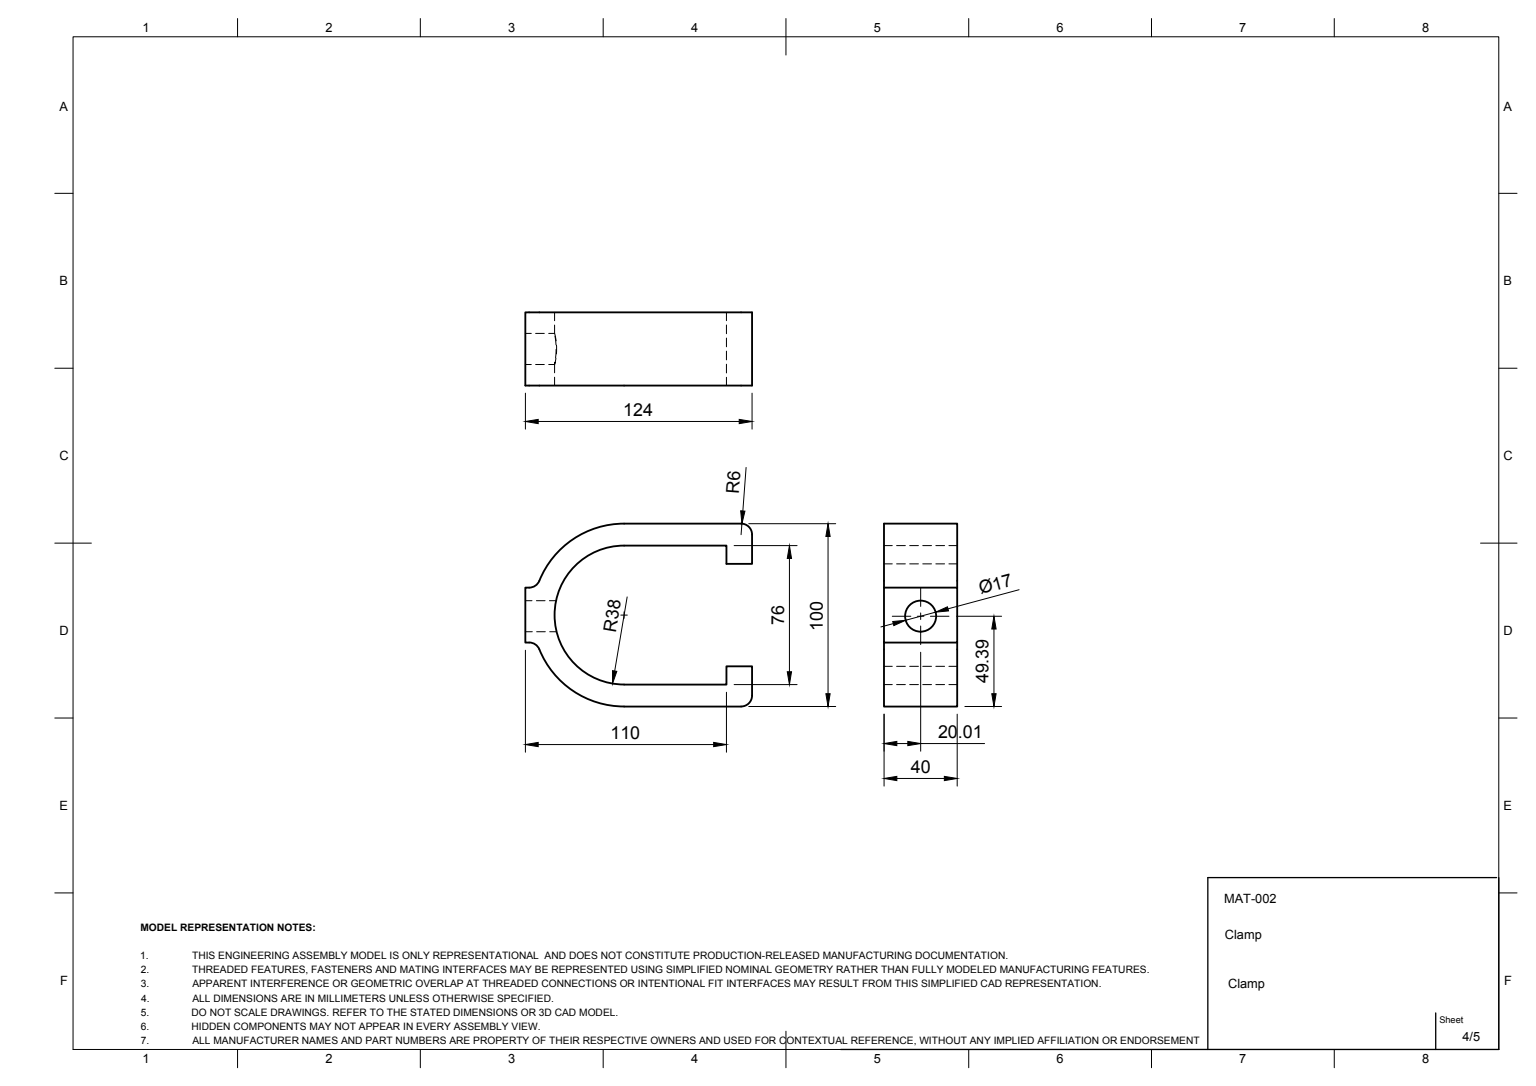
ISO-10303-21;
HEADER;
/* Generated by software containing ST-Developer
 * from STEP Tools, Inc. (www.steptools.com) 
 */

FILE_DESCRIPTION(
/* description */ ('STEP AP214'),
/* implementation_level */ '2;1');

FILE_NAME(
/* name */ 'Clamp.step',
/* time_stamp */ '2026-11-14T04:35:10-08:00',
/* author */ (''),
/* organization */ (''),
/* preprocessor_version */ 'ST-DEVELOPER v20.2',
/* originating_system */ 'Autodesk Translation Framework v15.17.0.0',
/* authorisation */ '');

FILE_SCHEMA (('AUTOMOTIVE_DESIGN { 1 0 10303 214 3 1 1 }'));
ENDSEC;

DATA;
#10=MECHANICAL_DESIGN_GEOMETRIC_PRESENTATION_REPRESENTATION('',(#108),#2477);
#47=FACE_BOUND('',#226,.T.);
#48=FACE_BOUND('',#235,.T.);
#50=CIRCLE('',#1508,8.49999999999998);
#51=CIRCLE('',#1512,38.);
#52=CIRCLE('',#1513,38.);
#53=CIRCLE('',#1520,50.);
#54=CIRCLE('',#1521,50.);
#55=CIRCLE('',#1526,50.);
#56=CIRCLE('',#1527,50.);
#57=CIRCLE('',#1532,6.);
#58=CIRCLE('',#1533,6.);
#59=CIRCLE('',#1534,6.);
#60=CIRCLE('',#1535,6.);
#61=CIRCLE('',#1537,6.);
#62=CIRCLE('',#1538,6.);
#63=CIRCLE('',#1539,6.);
#64=CIRCLE('',#1540,6.);
#86=B_SPLINE_CURVE_WITH_KNOTS('',3,(#2159,#2160,#2161,#2162,#2163,#2164,
#2165,#2166,#2167,#2168,#2169,#2170,#2171,#2172,#2173,#2174,#2175,#2176,
#2177),.UNSPECIFIED.,.F.,.F.,(4,2,2,2,3,2,2,2,4),(3.85552474626411,4.17737028900463,
4.49921583174514,4.82064221776852,5.14206860379189,5.46349498981527,5.78492137583865,
6.10676691857916,6.42861246131968),.UNSPECIFIED.);
#87=B_SPLINE_CURVE_WITH_KNOTS('',3,(#2181,#2182,#2183,#2184,#2185,#2186,
#2187,#2188,#2189,#2190,#2191,#2192,#2193,#2194,#2195,#2196,#2197,#2198),
 .UNSPECIFIED.,.F.,.F.,(4,2,2,2,2,2,2,2,4),(6.42861246131968,6.74954370836776,
7.07047495541584,7.39178893055184,7.71310290568784,8.03441688082384,8.35573085595985,
8.67666210300793,8.99759335005601),.UNSPECIFIED.);
#88=CYLINDRICAL_SURFACE('',#1507,8.49999999999998);
#89=CYLINDRICAL_SURFACE('',#1511,38.);
#90=CYLINDRICAL_SURFACE('',#1519,50.);
#91=CYLINDRICAL_SURFACE('',#1525,50.);
#92=CYLINDRICAL_SURFACE('',#1541,6.);
#93=CYLINDRICAL_SURFACE('',#1542,6.);
#94=CYLINDRICAL_SURFACE('',#1543,6.);
#95=CYLINDRICAL_SURFACE('',#1544,6.);
#100=SHAPE_REPRESENTATION_RELATIONSHIP('SRR','None',#2498,#104);
#104=ADVANCED_BREP_SHAPE_REPRESENTATION('',(#112),#2474);
#108=STYLED_ITEM('',(#2527),#112);
#112=MANIFOLD_SOLID_BREP('Body1',#1428);
#143=FACE_OUTER_BOUND('',#222,.T.);
#144=FACE_OUTER_BOUND('',#223,.T.);
#145=FACE_OUTER_BOUND('',#224,.T.);
#146=FACE_OUTER_BOUND('',#225,.T.);
#147=FACE_OUTER_BOUND('',#227,.T.);
#148=FACE_OUTER_BOUND('',#228,.T.);
#149=FACE_OUTER_BOUND('',#229,.T.);
#150=FACE_OUTER_BOUND('',#230,.T.);
#151=FACE_OUTER_BOUND('',#231,.T.);
#152=FACE_OUTER_BOUND('',#232,.T.);
#153=FACE_OUTER_BOUND('',#233,.T.);
#154=FACE_OUTER_BOUND('',#234,.T.);
#155=FACE_OUTER_BOUND('',#236,.T.);
#156=FACE_OUTER_BOUND('',#237,.T.);
#157=FACE_OUTER_BOUND('',#238,.T.);
#158=FACE_OUTER_BOUND('',#239,.T.);
#159=FACE_OUTER_BOUND('',#240,.T.);
#160=FACE_OUTER_BOUND('',#241,.T.);
#161=FACE_OUTER_BOUND('',#242,.T.);
#162=FACE_OUTER_BOUND('',#243,.T.);
#163=FACE_OUTER_BOUND('',#244,.T.);
#164=FACE_OUTER_BOUND('',#245,.T.);
#165=FACE_OUTER_BOUND('',#246,.T.);
#222=EDGE_LOOP('',(#1050,#1051,#1052,#1053,#1054));
#223=EDGE_LOOP('',(#1055,#1056,#1057,#1058));
#224=EDGE_LOOP('',(#1059,#1060,#1061,#1062));
#225=EDGE_LOOP('',(#1063,#1064,#1065,#1066));
#226=EDGE_LOOP('',(#1067,#1068));
#227=EDGE_LOOP('',(#1069,#1070,#1071,#1072));
#228=EDGE_LOOP('',(#1073,#1074,#1075,#1076));
#229=EDGE_LOOP('',(#1077,#1078,#1079,#1080));
#230=EDGE_LOOP('',(#1081,#1082,#1083,#1084));
#231=EDGE_LOOP('',(#1085,#1086,#1087,#1088));
#232=EDGE_LOOP('',(#1089,#1090,#1091,#1092));
#233=EDGE_LOOP('',(#1093,#1094,#1095,#1096));
#234=EDGE_LOOP('',(#1097,#1098,#1099,#1100));
#235=EDGE_LOOP('',(#1101));
#236=EDGE_LOOP('',(#1102,#1103,#1104,#1105));
#237=EDGE_LOOP('',(#1106,#1107,#1108,#1109));
#238=EDGE_LOOP('',(#1110,#1111,#1112,#1113));
#239=EDGE_LOOP('',(#1114,#1115,#1116,#1117));
#240=EDGE_LOOP('',(#1118,#1119,#1120,#1121));
#241=EDGE_LOOP('',(#1122,#1123,#1124,#1125,#1126,#1127,#1128,#1129,#1130,
#1131,#1132,#1133,#1134,#1135,#1136,#1137,#1138,#1139,#1140,#1141));
#242=EDGE_LOOP('',(#1142,#1143,#1144,#1145,#1146,#1147,#1148,#1149,#1150,
#1151,#1152,#1153,#1154,#1155,#1156,#1157,#1158,#1159,#1160,#1161));
#243=EDGE_LOOP('',(#1162,#1163,#1164,#1165));
#244=EDGE_LOOP('',(#1166,#1167,#1168,#1169));
#245=EDGE_LOOP('',(#1170,#1171,#1172,#1173));
#246=EDGE_LOOP('',(#1174,#1175,#1176,#1177));
#354=LINE('',#2179,#501);
#355=LINE('',#2202,#502);
#356=LINE('',#2204,#503);
#357=LINE('',#2206,#504);
#358=LINE('',#2207,#505);
#359=LINE('',#2210,#506);
#360=LINE('',#2212,#507);
#361=LINE('',#2213,#508);
#362=LINE('',#2218,#509);
#363=LINE('',#2222,#510);
#364=LINE('',#2224,#511);
#365=LINE('',#2225,#512);
#366=LINE('',#2228,#513);
#367=LINE('',#2230,#514);
#368=LINE('',#2231,#515);
#369=LINE('',#2234,#516);
#370=LINE('',#2236,#517);
#371=LINE('',#2237,#518);
#372=LINE('',#2240,#519);
#373=LINE('',#2242,#520);
#374=LINE('',#2243,#521);
#375=LINE('',#2247,#522);
#376=LINE('',#2249,#523);
#377=LINE('',#2251,#524);
#378=LINE('',#2252,#525);
#379=LINE('',#2257,#526);
#380=LINE('',#2262,#527);
#381=LINE('',#2264,#528);
#382=LINE('',#2266,#529);
#383=LINE('',#2267,#530);
#384=LINE('',#2270,#531);
#385=LINE('',#2272,#532);
#386=LINE('',#2273,#533);
#387=LINE('',#2276,#534);
#388=LINE('',#2278,#535);
#389=LINE('',#2279,#536);
#390=LINE('',#2285,#537);
#391=LINE('',#2288,#538);
#392=LINE('',#2291,#539);
#393=LINE('',#2293,#540);
#394=LINE('',#2294,#541);
#395=LINE('',#2298,#542);
#396=LINE('',#2300,#543);
#397=LINE('',#2302,#544);
#398=LINE('',#2303,#545);
#399=LINE('',#2305,#546);
#400=LINE('',#2306,#547);
#501=VECTOR('',#1742,8.49999999999998);
#502=VECTOR('',#1747,1000.);
#503=VECTOR('',#1748,1000.);
#504=VECTOR('',#1749,1000.);
#505=VECTOR('',#1750,1000.);
#506=VECTOR('',#1753,1000.);
#507=VECTOR('',#1754,1000.);
#508=VECTOR('',#1755,1000.);
#509=VECTOR('',#1760,1000.);
#510=VECTOR('',#1765,1000.);
#511=VECTOR('',#1766,1000.);
#512=VECTOR('',#1767,1000.);
#513=VECTOR('',#1770,1000.);
#514=VECTOR('',#1771,1000.);
#515=VECTOR('',#1772,1000.);
#516=VECTOR('',#1775,1000.);
#517=VECTOR('',#1776,1000.);
#518=VECTOR('',#1777,1000.);
#519=VECTOR('',#1780,1000.);
#520=VECTOR('',#1781,1000.);
#521=VECTOR('',#1782,1000.);
#522=VECTOR('',#1785,1000.);
#523=VECTOR('',#1786,1000.);
#524=VECTOR('',#1787,1000.);
#525=VECTOR('',#1788,1000.);
#526=VECTOR('',#1793,1000.);
#527=VECTOR('',#1798,1000.);
#528=VECTOR('',#1799,1000.);
#529=VECTOR('',#1800,1000.);
#530=VECTOR('',#1801,1000.);
#531=VECTOR('',#1804,1000.);
#532=VECTOR('',#1805,1000.);
#533=VECTOR('',#1806,1000.);
#534=VECTOR('',#1809,1000.);
#535=VECTOR('',#1810,1000.);
#536=VECTOR('',#1811,1000.);
#537=VECTOR('',#1816,1000.);
#538=VECTOR('',#1819,1000.);
#539=VECTOR('',#1822,1000.);
#540=VECTOR('',#1823,1000.);
#541=VECTOR('',#1824,1000.);
#542=VECTOR('',#1827,1000.);
#543=VECTOR('',#1828,1000.);
#544=VECTOR('',#1829,1000.);
#545=VECTOR('',#1830,1000.);
#546=VECTOR('',#1833,1000.);
#547=VECTOR('',#1834,1000.);
#622=VERTEX_POINT('',#2157);
#623=VERTEX_POINT('',#2158);
#624=VERTEX_POINT('',#2178);
#625=VERTEX_POINT('',#2200);
#626=VERTEX_POINT('',#2201);
#627=VERTEX_POINT('',#2203);
#628=VERTEX_POINT('',#2205);
#629=VERTEX_POINT('',#2209);
#630=VERTEX_POINT('',#2211);
#631=VERTEX_POINT('',#2215);
#632=VERTEX_POINT('',#2217);
#633=VERTEX_POINT('',#2221);
#634=VERTEX_POINT('',#2223);
#635=VERTEX_POINT('',#2227);
#636=VERTEX_POINT('',#2229);
#637=VERTEX_POINT('',#2233);
#638=VERTEX_POINT('',#2235);
#639=VERTEX_POINT('',#2239);
#640=VERTEX_POINT('',#2241);
#641=VERTEX_POINT('',#2245);
#642=VERTEX_POINT('',#2246);
#643=VERTEX_POINT('',#2248);
#644=VERTEX_POINT('',#2250);
#645=VERTEX_POINT('',#2254);
#646=VERTEX_POINT('',#2256);
#647=VERTEX_POINT('',#2260);
#648=VERTEX_POINT('',#2261);
#649=VERTEX_POINT('',#2263);
#650=VERTEX_POINT('',#2265);
#651=VERTEX_POINT('',#2269);
#652=VERTEX_POINT('',#2271);
#653=VERTEX_POINT('',#2275);
#654=VERTEX_POINT('',#2277);
#655=VERTEX_POINT('',#2281);
#656=VERTEX_POINT('',#2282);
#657=VERTEX_POINT('',#2284);
#658=VERTEX_POINT('',#2286);
#659=VERTEX_POINT('',#2290);
#660=VERTEX_POINT('',#2292);
#661=VERTEX_POINT('',#2296);
#662=VERTEX_POINT('',#2297);
#663=VERTEX_POINT('',#2299);
#664=VERTEX_POINT('',#2301);
#775=EDGE_CURVE('',#622,#623,#86,.T.);
#776=EDGE_CURVE('',#623,#624,#354,.T.);
#777=EDGE_CURVE('',#624,#624,#50,.T.);
#778=EDGE_CURVE('',#623,#622,#87,.T.);
#779=EDGE_CURVE('',#625,#626,#355,.T.);
#780=EDGE_CURVE('',#627,#625,#356,.T.);
#781=EDGE_CURVE('',#627,#628,#357,.T.);
#782=EDGE_CURVE('',#628,#626,#358,.T.);
#783=EDGE_CURVE('',#629,#625,#359,.T.);
#784=EDGE_CURVE('',#630,#629,#360,.T.);
#785=EDGE_CURVE('',#630,#627,#361,.T.);
#786=EDGE_CURVE('',#631,#629,#51,.T.);
#787=EDGE_CURVE('',#632,#631,#362,.T.);
#788=EDGE_CURVE('',#632,#630,#52,.T.);
#789=EDGE_CURVE('',#633,#631,#363,.T.);
#790=EDGE_CURVE('',#634,#633,#364,.T.);
#791=EDGE_CURVE('',#634,#632,#365,.T.);
#792=EDGE_CURVE('',#635,#633,#366,.T.);
#793=EDGE_CURVE('',#636,#635,#367,.T.);
#794=EDGE_CURVE('',#636,#634,#368,.T.);
#795=EDGE_CURVE('',#637,#635,#369,.T.);
#796=EDGE_CURVE('',#638,#637,#370,.T.);
#797=EDGE_CURVE('',#638,#636,#371,.T.);
#798=EDGE_CURVE('',#639,#637,#372,.T.);
#799=EDGE_CURVE('',#639,#640,#373,.T.);
#800=EDGE_CURVE('',#640,#638,#374,.T.);
#801=EDGE_CURVE('',#641,#642,#375,.T.);
#802=EDGE_CURVE('',#642,#643,#376,.T.);
#803=EDGE_CURVE('',#644,#643,#377,.T.);
#804=EDGE_CURVE('',#641,#644,#378,.T.);
#805=EDGE_CURVE('',#645,#644,#53,.T.);
#806=EDGE_CURVE('',#645,#646,#379,.T.);
#807=EDGE_CURVE('',#646,#641,#54,.T.);
#808=EDGE_CURVE('',#647,#648,#380,.T.);
#809=EDGE_CURVE('',#648,#649,#381,.T.);
#810=EDGE_CURVE('',#650,#649,#382,.T.);
#811=EDGE_CURVE('',#647,#650,#383,.T.);
#812=EDGE_CURVE('',#651,#650,#384,.T.);
#813=EDGE_CURVE('',#652,#651,#385,.T.);
#814=EDGE_CURVE('',#652,#647,#386,.T.);
#815=EDGE_CURVE('',#653,#651,#387,.T.);
#816=EDGE_CURVE('',#653,#654,#388,.T.);
#817=EDGE_CURVE('',#654,#652,#389,.T.);
#818=EDGE_CURVE('',#655,#656,#55,.T.);
#819=EDGE_CURVE('',#656,#657,#390,.T.);
#820=EDGE_CURVE('',#658,#657,#56,.T.);
#821=EDGE_CURVE('',#655,#658,#391,.T.);
#822=EDGE_CURVE('',#659,#658,#392,.T.);
#823=EDGE_CURVE('',#659,#660,#393,.T.);
#824=EDGE_CURVE('',#660,#655,#394,.T.);
#825=EDGE_CURVE('',#661,#662,#395,.T.);
#826=EDGE_CURVE('',#662,#663,#396,.T.);
#827=EDGE_CURVE('',#664,#663,#397,.T.);
#828=EDGE_CURVE('',#661,#664,#398,.T.);
#829=EDGE_CURVE('',#626,#664,#399,.T.);
#830=EDGE_CURVE('',#628,#661,#400,.T.);
#831=EDGE_CURVE('',#660,#662,#57,.T.);
#832=EDGE_CURVE('',#640,#642,#58,.T.);
#833=EDGE_CURVE('',#646,#648,#59,.T.);
#834=EDGE_CURVE('',#654,#656,#60,.T.);
#835=EDGE_CURVE('',#663,#659,#61,.T.);
#836=EDGE_CURVE('',#657,#653,#62,.T.);
#837=EDGE_CURVE('',#649,#645,#63,.T.);
#838=EDGE_CURVE('',#643,#639,#64,.T.);
#1050=ORIENTED_EDGE('',*,*,#775,.T.);
#1051=ORIENTED_EDGE('',*,*,#776,.T.);
#1052=ORIENTED_EDGE('',*,*,#777,.T.);
#1053=ORIENTED_EDGE('',*,*,#776,.F.);
#1054=ORIENTED_EDGE('',*,*,#778,.T.);
#1055=ORIENTED_EDGE('',*,*,#779,.F.);
#1056=ORIENTED_EDGE('',*,*,#780,.F.);
#1057=ORIENTED_EDGE('',*,*,#781,.T.);
#1058=ORIENTED_EDGE('',*,*,#782,.T.);
#1059=ORIENTED_EDGE('',*,*,#783,.F.);
#1060=ORIENTED_EDGE('',*,*,#784,.F.);
#1061=ORIENTED_EDGE('',*,*,#785,.T.);
#1062=ORIENTED_EDGE('',*,*,#780,.T.);
#1063=ORIENTED_EDGE('',*,*,#786,.F.);
#1064=ORIENTED_EDGE('',*,*,#787,.F.);
#1065=ORIENTED_EDGE('',*,*,#788,.T.);
#1066=ORIENTED_EDGE('',*,*,#784,.T.);
#1067=ORIENTED_EDGE('',*,*,#775,.F.);
#1068=ORIENTED_EDGE('',*,*,#778,.F.);
#1069=ORIENTED_EDGE('',*,*,#789,.F.);
#1070=ORIENTED_EDGE('',*,*,#790,.F.);
#1071=ORIENTED_EDGE('',*,*,#791,.T.);
#1072=ORIENTED_EDGE('',*,*,#787,.T.);
#1073=ORIENTED_EDGE('',*,*,#792,.F.);
#1074=ORIENTED_EDGE('',*,*,#793,.F.);
#1075=ORIENTED_EDGE('',*,*,#794,.T.);
#1076=ORIENTED_EDGE('',*,*,#790,.T.);
#1077=ORIENTED_EDGE('',*,*,#795,.F.);
#1078=ORIENTED_EDGE('',*,*,#796,.F.);
#1079=ORIENTED_EDGE('',*,*,#797,.T.);
#1080=ORIENTED_EDGE('',*,*,#793,.T.);
#1081=ORIENTED_EDGE('',*,*,#798,.F.);
#1082=ORIENTED_EDGE('',*,*,#799,.T.);
#1083=ORIENTED_EDGE('',*,*,#800,.T.);
#1084=ORIENTED_EDGE('',*,*,#796,.T.);
#1085=ORIENTED_EDGE('',*,*,#801,.T.);
#1086=ORIENTED_EDGE('',*,*,#802,.T.);
#1087=ORIENTED_EDGE('',*,*,#803,.F.);
#1088=ORIENTED_EDGE('',*,*,#804,.F.);
#1089=ORIENTED_EDGE('',*,*,#805,.F.);
#1090=ORIENTED_EDGE('',*,*,#806,.T.);
#1091=ORIENTED_EDGE('',*,*,#807,.T.);
#1092=ORIENTED_EDGE('',*,*,#804,.T.);
#1093=ORIENTED_EDGE('',*,*,#808,.T.);
#1094=ORIENTED_EDGE('',*,*,#809,.T.);
#1095=ORIENTED_EDGE('',*,*,#810,.F.);
#1096=ORIENTED_EDGE('',*,*,#811,.F.);
#1097=ORIENTED_EDGE('',*,*,#812,.F.);
#1098=ORIENTED_EDGE('',*,*,#813,.F.);
#1099=ORIENTED_EDGE('',*,*,#814,.T.);
#1100=ORIENTED_EDGE('',*,*,#811,.T.);
#1101=ORIENTED_EDGE('',*,*,#777,.F.);
#1102=ORIENTED_EDGE('',*,*,#815,.F.);
#1103=ORIENTED_EDGE('',*,*,#816,.T.);
#1104=ORIENTED_EDGE('',*,*,#817,.T.);
#1105=ORIENTED_EDGE('',*,*,#813,.T.);
#1106=ORIENTED_EDGE('',*,*,#818,.T.);
#1107=ORIENTED_EDGE('',*,*,#819,.T.);
#1108=ORIENTED_EDGE('',*,*,#820,.F.);
#1109=ORIENTED_EDGE('',*,*,#821,.F.);
#1110=ORIENTED_EDGE('',*,*,#822,.F.);
#1111=ORIENTED_EDGE('',*,*,#823,.T.);
#1112=ORIENTED_EDGE('',*,*,#824,.T.);
#1113=ORIENTED_EDGE('',*,*,#821,.T.);
#1114=ORIENTED_EDGE('',*,*,#825,.T.);
#1115=ORIENTED_EDGE('',*,*,#826,.T.);
#1116=ORIENTED_EDGE('',*,*,#827,.F.);
#1117=ORIENTED_EDGE('',*,*,#828,.F.);
#1118=ORIENTED_EDGE('',*,*,#829,.F.);
#1119=ORIENTED_EDGE('',*,*,#782,.F.);
#1120=ORIENTED_EDGE('',*,*,#830,.T.);
#1121=ORIENTED_EDGE('',*,*,#828,.T.);
#1122=ORIENTED_EDGE('',*,*,#824,.F.);
#1123=ORIENTED_EDGE('',*,*,#831,.T.);
#1124=ORIENTED_EDGE('',*,*,#825,.F.);
#1125=ORIENTED_EDGE('',*,*,#830,.F.);
#1126=ORIENTED_EDGE('',*,*,#781,.F.);
#1127=ORIENTED_EDGE('',*,*,#785,.F.);
#1128=ORIENTED_EDGE('',*,*,#788,.F.);
#1129=ORIENTED_EDGE('',*,*,#791,.F.);
#1130=ORIENTED_EDGE('',*,*,#794,.F.);
#1131=ORIENTED_EDGE('',*,*,#797,.F.);
#1132=ORIENTED_EDGE('',*,*,#800,.F.);
#1133=ORIENTED_EDGE('',*,*,#832,.T.);
#1134=ORIENTED_EDGE('',*,*,#801,.F.);
#1135=ORIENTED_EDGE('',*,*,#807,.F.);
#1136=ORIENTED_EDGE('',*,*,#833,.T.);
#1137=ORIENTED_EDGE('',*,*,#808,.F.);
#1138=ORIENTED_EDGE('',*,*,#814,.F.);
#1139=ORIENTED_EDGE('',*,*,#817,.F.);
#1140=ORIENTED_EDGE('',*,*,#834,.T.);
#1141=ORIENTED_EDGE('',*,*,#818,.F.);
#1142=ORIENTED_EDGE('',*,*,#827,.T.);
#1143=ORIENTED_EDGE('',*,*,#835,.T.);
#1144=ORIENTED_EDGE('',*,*,#822,.T.);
#1145=ORIENTED_EDGE('',*,*,#820,.T.);
#1146=ORIENTED_EDGE('',*,*,#836,.T.);
#1147=ORIENTED_EDGE('',*,*,#815,.T.);
#1148=ORIENTED_EDGE('',*,*,#812,.T.);
#1149=ORIENTED_EDGE('',*,*,#810,.T.);
#1150=ORIENTED_EDGE('',*,*,#837,.T.);
#1151=ORIENTED_EDGE('',*,*,#805,.T.);
#1152=ORIENTED_EDGE('',*,*,#803,.T.);
#1153=ORIENTED_EDGE('',*,*,#838,.T.);
#1154=ORIENTED_EDGE('',*,*,#798,.T.);
#1155=ORIENTED_EDGE('',*,*,#795,.T.);
#1156=ORIENTED_EDGE('',*,*,#792,.T.);
#1157=ORIENTED_EDGE('',*,*,#789,.T.);
#1158=ORIENTED_EDGE('',*,*,#786,.T.);
#1159=ORIENTED_EDGE('',*,*,#783,.T.);
#1160=ORIENTED_EDGE('',*,*,#779,.T.);
#1161=ORIENTED_EDGE('',*,*,#829,.T.);
#1162=ORIENTED_EDGE('',*,*,#831,.F.);
#1163=ORIENTED_EDGE('',*,*,#823,.F.);
#1164=ORIENTED_EDGE('',*,*,#835,.F.);
#1165=ORIENTED_EDGE('',*,*,#826,.F.);
#1166=ORIENTED_EDGE('',*,*,#832,.F.);
#1167=ORIENTED_EDGE('',*,*,#799,.F.);
#1168=ORIENTED_EDGE('',*,*,#838,.F.);
#1169=ORIENTED_EDGE('',*,*,#802,.F.);
#1170=ORIENTED_EDGE('',*,*,#833,.F.);
#1171=ORIENTED_EDGE('',*,*,#806,.F.);
#1172=ORIENTED_EDGE('',*,*,#837,.F.);
#1173=ORIENTED_EDGE('',*,*,#809,.F.);
#1174=ORIENTED_EDGE('',*,*,#834,.F.);
#1175=ORIENTED_EDGE('',*,*,#816,.F.);
#1176=ORIENTED_EDGE('',*,*,#836,.F.);
#1177=ORIENTED_EDGE('',*,*,#819,.F.);
#1316=PLANE('',#1509);
#1317=PLANE('',#1510);
#1318=PLANE('',#1514);
#1319=PLANE('',#1515);
#1320=PLANE('',#1516);
#1321=PLANE('',#1517);
#1322=PLANE('',#1518);
#1323=PLANE('',#1522);
#1324=PLANE('',#1523);
#1325=PLANE('',#1524);
#1326=PLANE('',#1528);
#1327=PLANE('',#1529);
#1328=PLANE('',#1530);
#1329=PLANE('',#1531);
#1330=PLANE('',#1536);
#1376=ADVANCED_FACE('',(#143),#88,.F.);
#1377=ADVANCED_FACE('',(#144),#1316,.T.);
#1378=ADVANCED_FACE('',(#145),#1317,.T.);
#1379=ADVANCED_FACE('',(#146,#47),#89,.F.);
#1380=ADVANCED_FACE('',(#147),#1318,.T.);
#1381=ADVANCED_FACE('',(#148),#1319,.T.);
#1382=ADVANCED_FACE('',(#149),#1320,.T.);
#1383=ADVANCED_FACE('',(#150),#1321,.T.);
#1384=ADVANCED_FACE('',(#151),#1322,.T.);
#1385=ADVANCED_FACE('',(#152),#90,.T.);
#1386=ADVANCED_FACE('',(#153),#1323,.T.);
#1387=ADVANCED_FACE('',(#154,#48),#1324,.T.);
#1388=ADVANCED_FACE('',(#155),#1325,.T.);
#1389=ADVANCED_FACE('',(#156),#91,.T.);
#1390=ADVANCED_FACE('',(#157),#1326,.T.);
#1391=ADVANCED_FACE('',(#158),#1327,.T.);
#1392=ADVANCED_FACE('',(#159),#1328,.T.);
#1393=ADVANCED_FACE('',(#160),#1329,.F.);
#1394=ADVANCED_FACE('',(#161),#1330,.T.);
#1395=ADVANCED_FACE('',(#162),#92,.T.);
#1396=ADVANCED_FACE('',(#163),#93,.T.);
#1397=ADVANCED_FACE('',(#164),#94,.F.);
#1398=ADVANCED_FACE('',(#165),#95,.F.);
#1428=CLOSED_SHELL('',(#1376,#1377,#1378,#1379,#1380,#1381,#1382,#1383,
#1384,#1385,#1386,#1387,#1388,#1389,#1390,#1391,#1392,#1393,#1394,#1395,
#1396,#1397,#1398));
#1506=AXIS2_PLACEMENT_3D('',#2155,#1738,#1739);
#1507=AXIS2_PLACEMENT_3D('',#2156,#1740,#1741);
#1508=AXIS2_PLACEMENT_3D('',#2180,#1743,#1744);
#1509=AXIS2_PLACEMENT_3D('',#2199,#1745,#1746);
#1510=AXIS2_PLACEMENT_3D('',#2208,#1751,#1752);
#1511=AXIS2_PLACEMENT_3D('',#2214,#1756,#1757);
#1512=AXIS2_PLACEMENT_3D('',#2216,#1758,#1759);
#1513=AXIS2_PLACEMENT_3D('',#2219,#1761,#1762);
#1514=AXIS2_PLACEMENT_3D('',#2220,#1763,#1764);
#1515=AXIS2_PLACEMENT_3D('',#2226,#1768,#1769);
#1516=AXIS2_PLACEMENT_3D('',#2232,#1773,#1774);
#1517=AXIS2_PLACEMENT_3D('',#2238,#1778,#1779);
#1518=AXIS2_PLACEMENT_3D('',#2244,#1783,#1784);
#1519=AXIS2_PLACEMENT_3D('',#2253,#1789,#1790);
#1520=AXIS2_PLACEMENT_3D('',#2255,#1791,#1792);
#1521=AXIS2_PLACEMENT_3D('',#2258,#1794,#1795);
#1522=AXIS2_PLACEMENT_3D('',#2259,#1796,#1797);
#1523=AXIS2_PLACEMENT_3D('',#2268,#1802,#1803);
#1524=AXIS2_PLACEMENT_3D('',#2274,#1807,#1808);
#1525=AXIS2_PLACEMENT_3D('',#2280,#1812,#1813);
#1526=AXIS2_PLACEMENT_3D('',#2283,#1814,#1815);
#1527=AXIS2_PLACEMENT_3D('',#2287,#1817,#1818);
#1528=AXIS2_PLACEMENT_3D('',#2289,#1820,#1821);
#1529=AXIS2_PLACEMENT_3D('',#2295,#1825,#1826);
#1530=AXIS2_PLACEMENT_3D('',#2304,#1831,#1832);
#1531=AXIS2_PLACEMENT_3D('',#2307,#1835,#1836);
#1532=AXIS2_PLACEMENT_3D('',#2308,#1837,#1838);
#1533=AXIS2_PLACEMENT_3D('',#2309,#1839,#1840);
#1534=AXIS2_PLACEMENT_3D('',#2310,#1841,#1842);
#1535=AXIS2_PLACEMENT_3D('',#2311,#1843,#1844);
#1536=AXIS2_PLACEMENT_3D('',#2312,#1845,#1846);
#1537=AXIS2_PLACEMENT_3D('',#2313,#1847,#1848);
#1538=AXIS2_PLACEMENT_3D('',#2314,#1849,#1850);
#1539=AXIS2_PLACEMENT_3D('',#2315,#1851,#1852);
#1540=AXIS2_PLACEMENT_3D('',#2316,#1853,#1854);
#1541=AXIS2_PLACEMENT_3D('',#2317,#1855,#1856);
#1542=AXIS2_PLACEMENT_3D('',#2318,#1857,#1858);
#1543=AXIS2_PLACEMENT_3D('',#2319,#1859,#1860);
#1544=AXIS2_PLACEMENT_3D('',#2320,#1861,#1862);
#1738=DIRECTION('axis',(0.,0.,1.));
#1739=DIRECTION('refdir',(1.,0.,0.));
#1740=DIRECTION('center_axis',(0.,1.,0.));
#1741=DIRECTION('ref_axis',(0.,0.,1.));
#1742=DIRECTION('',(0.,1.,0.));
#1743=DIRECTION('center_axis',(0.,1.,0.));
#1744=DIRECTION('ref_axis',(0.,0.,1.));
#1745=DIRECTION('center_axis',(0.,1.,0.));
#1746=DIRECTION('ref_axis',(0.,0.,1.));
#1747=DIRECTION('',(-1.,0.,0.));
#1748=DIRECTION('',(0.,0.,1.));
#1749=DIRECTION('',(-1.,0.,0.));
#1750=DIRECTION('',(0.,0.,1.));
#1751=DIRECTION('center_axis',(-1.,-2.47817639425258E-16,0.));
#1752=DIRECTION('ref_axis',(2.47817639425258E-16,-1.,0.));
#1753=DIRECTION('',(2.47817639425258E-16,-1.,0.));
#1754=DIRECTION('',(0.,0.,1.));
#1755=DIRECTION('',(2.47817639425258E-16,-1.,0.));
#1756=DIRECTION('center_axis',(0.,0.,1.));
#1757=DIRECTION('ref_axis',(1.,0.,0.));
#1758=DIRECTION('center_axis',(0.,0.,-1.));
#1759=DIRECTION('ref_axis',(1.,0.,0.));
#1760=DIRECTION('',(0.,0.,1.));
#1761=DIRECTION('center_axis',(0.,0.,-1.));
#1762=DIRECTION('ref_axis',(1.,0.,0.));
#1763=DIRECTION('center_axis',(1.,0.,0.));
#1764=DIRECTION('ref_axis',(0.,0.,-1.));
#1765=DIRECTION('',(0.,1.,0.));
#1766=DIRECTION('',(0.,0.,1.));
#1767=DIRECTION('',(0.,1.,0.));
#1768=DIRECTION('center_axis',(0.,1.,0.));
#1769=DIRECTION('ref_axis',(0.,0.,1.));
#1770=DIRECTION('',(-1.,0.,0.));
#1771=DIRECTION('',(0.,0.,1.));
#1772=DIRECTION('',(-1.,0.,0.));
#1773=DIRECTION('center_axis',(1.,0.,0.));
#1774=DIRECTION('ref_axis',(0.,0.,-1.));
#1775=DIRECTION('',(0.,1.,0.));
#1776=DIRECTION('',(0.,0.,1.));
#1777=DIRECTION('',(0.,1.,0.));
#1778=DIRECTION('center_axis',(0.,-1.,0.));
#1779=DIRECTION('ref_axis',(0.,0.,-1.));
#1780=DIRECTION('',(1.,0.,0.));
#1781=DIRECTION('',(0.,0.,-1.));
#1782=DIRECTION('',(1.,0.,0.));
#1783=DIRECTION('center_axis',(-1.,-9.91270557701033E-17,0.));
#1784=DIRECTION('ref_axis',(9.91270557701033E-17,-1.,0.));
#1785=DIRECTION('',(9.91270557701033E-17,-1.,0.));
#1786=DIRECTION('',(0.,0.,1.));
#1787=DIRECTION('',(9.91270557701033E-17,-1.,0.));
#1788=DIRECTION('',(0.,0.,1.));
#1789=DIRECTION('center_axis',(0.,0.,1.));
#1790=DIRECTION('ref_axis',(1.,0.,0.));
#1791=DIRECTION('center_axis',(0.,0.,1.));
#1792=DIRECTION('ref_axis',(1.,0.,0.));
#1793=DIRECTION('',(0.,0.,-1.));
#1794=DIRECTION('center_axis',(0.,0.,1.));
#1795=DIRECTION('ref_axis',(1.,0.,0.));
#1796=DIRECTION('center_axis',(-1.,0.,0.));
#1797=DIRECTION('ref_axis',(0.,0.,1.));
#1798=DIRECTION('',(0.,-1.,0.));
#1799=DIRECTION('',(0.,0.,1.));
#1800=DIRECTION('',(0.,-1.,0.));
#1801=DIRECTION('',(0.,0.,1.));
#1802=DIRECTION('center_axis',(0.,1.,0.));
#1803=DIRECTION('ref_axis',(0.,0.,1.));
#1804=DIRECTION('',(-1.,0.,0.));
#1805=DIRECTION('',(0.,0.,1.));
#1806=DIRECTION('',(-1.,0.,0.));
#1807=DIRECTION('center_axis',(1.,0.,0.));
#1808=DIRECTION('ref_axis',(0.,0.,-1.));
#1809=DIRECTION('',(0.,1.,0.));
#1810=DIRECTION('',(0.,0.,-1.));
#1811=DIRECTION('',(0.,1.,0.));
#1812=DIRECTION('center_axis',(0.,0.,1.));
#1813=DIRECTION('ref_axis',(1.,0.,0.));
#1814=DIRECTION('center_axis',(0.,0.,1.));
#1815=DIRECTION('ref_axis',(1.,0.,0.));
#1816=DIRECTION('',(0.,0.,1.));
#1817=DIRECTION('center_axis',(0.,0.,1.));
#1818=DIRECTION('ref_axis',(1.,0.,0.));
#1819=DIRECTION('',(0.,0.,1.));
#1820=DIRECTION('center_axis',(1.,0.,0.));
#1821=DIRECTION('ref_axis',(0.,0.,-1.));
#1822=DIRECTION('',(0.,1.,0.));
#1823=DIRECTION('',(0.,0.,-1.));
#1824=DIRECTION('',(0.,1.,0.));
#1825=DIRECTION('center_axis',(0.,-1.,0.));
#1826=DIRECTION('ref_axis',(0.,0.,-1.));
#1827=DIRECTION('',(1.,0.,0.));
#1828=DIRECTION('',(0.,0.,1.));
#1829=DIRECTION('',(1.,0.,0.));
#1830=DIRECTION('',(0.,0.,1.));
#1831=DIRECTION('center_axis',(-1.,0.,0.));
#1832=DIRECTION('ref_axis',(0.,0.,1.));
#1833=DIRECTION('',(0.,-1.,0.));
#1834=DIRECTION('',(0.,-1.,0.));
#1835=DIRECTION('center_axis',(0.,0.,1.));
#1836=DIRECTION('ref_axis',(1.,0.,0.));
#1837=DIRECTION('center_axis',(0.,0.,-1.));
#1838=DIRECTION('ref_axis',(1.,0.,0.));
#1839=DIRECTION('center_axis',(0.,0.,-1.));
#1840=DIRECTION('ref_axis',(1.,0.,0.));
#1841=DIRECTION('center_axis',(0.,0.,1.));
#1842=DIRECTION('ref_axis',(1.,0.,0.));
#1843=DIRECTION('center_axis',(0.,0.,1.));
#1844=DIRECTION('ref_axis',(1.,0.,0.));
#1845=DIRECTION('center_axis',(0.,0.,1.));
#1846=DIRECTION('ref_axis',(1.,0.,0.));
#1847=DIRECTION('center_axis',(0.,0.,1.));
#1848=DIRECTION('ref_axis',(1.,0.,0.));
#1849=DIRECTION('center_axis',(0.,0.,-1.));
#1850=DIRECTION('ref_axis',(1.,0.,0.));
#1851=DIRECTION('center_axis',(0.,0.,-1.));
#1852=DIRECTION('ref_axis',(1.,0.,0.));
#1853=DIRECTION('center_axis',(0.,0.,1.));
#1854=DIRECTION('ref_axis',(1.,0.,0.));
#1855=DIRECTION('center_axis',(0.,0.,1.));
#1856=DIRECTION('ref_axis',(1.,0.,0.));
#1857=DIRECTION('center_axis',(0.,0.,1.));
#1858=DIRECTION('ref_axis',(1.,0.,0.));
#1859=DIRECTION('center_axis',(0.,0.,1.));
#1860=DIRECTION('ref_axis',(1.,0.,0.));
#1861=DIRECTION('center_axis',(0.,0.,1.));
#1862=DIRECTION('ref_axis',(1.,0.,0.));
#2155=CARTESIAN_POINT('',(0.,0.,0.));
#2156=CARTESIAN_POINT('Origin',(-0.619834889991667,57.4408918778678,-9.99053328739284));
#2157=CARTESIAN_POINT('',(-0.619834889991667,41.4359646982476,-1.49053328739287));
#2158=CARTESIAN_POINT('',(-0.619834889991667,41.4359646982476,-18.4905332873928));
#2159=CARTESIAN_POINT('Ctrl Pts',(-0.619834889991664,41.4359646982476,-1.49053328739287));
#2160=CARTESIAN_POINT('Ctrl Pts',(-1.69251426133731,41.4186890416464,-1.49053328739286));
#2161=CARTESIAN_POINT('Ctrl Pts',(-2.83333550672754,41.3503146663282,-1.70589301181152));
#2162=CARTESIAN_POINT('Ctrl Pts',(-4.92696200368771,41.1358561238382,-2.57544700481013));
#2163=CARTESIAN_POINT('Ctrl Pts',(-5.880109476723,40.9922072228327,-3.22941616388057));
#2164=CARTESIAN_POINT('Ctrl Pts',(-7.38400452652566,40.7259525153024,-4.73446508972372));
#2165=CARTESIAN_POINT('Ctrl Pts',(-8.03690297146328,40.5856574031577,-5.68707722694506));
#2166=CARTESIAN_POINT('Ctrl Pts',(-8.90492499084854,40.387359614178,-7.77921932756061));
#2167=CARTESIAN_POINT('Ctrl Pts',(-9.11983488999165,40.332259216097,-8.91911200064825));
#2168=CARTESIAN_POINT('Ctrl Pts',(-9.11983488999165,40.332259216097,-9.99053328739285));
#2169=CARTESIAN_POINT('Ctrl Pts',(-9.11983488999165,40.332259216097,-11.0619545741374));
#2170=CARTESIAN_POINT('Ctrl Pts',(-8.90492499084854,40.387359614178,-12.2018472472251));
#2171=CARTESIAN_POINT('Ctrl Pts',(-8.03690297146328,40.5856574031577,-14.2939893478406));
#2172=CARTESIAN_POINT('Ctrl Pts',(-7.38400452652566,40.7259525153024,-15.246601485062));
#2173=CARTESIAN_POINT('Ctrl Pts',(-5.880109476723,40.9922072228327,-16.7516504109051));
#2174=CARTESIAN_POINT('Ctrl Pts',(-4.92696200368771,41.1358561238382,-17.4056195699756));
#2175=CARTESIAN_POINT('Ctrl Pts',(-2.83333550672754,41.3503146663282,-18.2751735629742));
#2176=CARTESIAN_POINT('Ctrl Pts',(-1.69251426133732,41.4186890416464,-18.4905332873928));
#2177=CARTESIAN_POINT('Ctrl Pts',(-0.619834889991667,41.4359646982476,-18.4905332873928));
#2178=CARTESIAN_POINT('',(-0.619834889991668,57.4408918778678,-18.4905332873928));
#2179=CARTESIAN_POINT('',(-0.619834889991668,57.4408918778678,-18.4905332873928));
#2180=CARTESIAN_POINT('Origin',(-0.619834889991667,57.4408918778678,-9.99053328739284));
#2181=CARTESIAN_POINT('Ctrl Pts',(-0.619834889991667,41.4359646982476,-18.4905332873928));
#2182=CARTESIAN_POINT('Ctrl Pts',(0.449797224212465,41.4531912783312,-18.4905332873928));
#2183=CARTESIAN_POINT('Ctrl Pts',(1.5892054277245,41.4218020260498,-18.2762675827069));
#2184=CARTESIAN_POINT('Ctrl Pts',(3.68206578130104,41.2758539577384,-17.4085452787979));
#2185=CARTESIAN_POINT('Ctrl Pts',(4.63575860476113,41.1637585877487,-16.755256589616));
#2186=CARTESIAN_POINT('Ctrl Pts',(6.14230817135067,40.9476179603983,-15.2497032680988));
#2187=CARTESIAN_POINT('Ctrl Pts',(6.79640351541145,40.8293540083924,-14.2956842723128));
#2188=CARTESIAN_POINT('Ctrl Pts',(7.66541391347513,40.6607235779339,-12.2017692944875));
#2189=CARTESIAN_POINT('Ctrl Pts',(7.88016511000832,40.6131682833795,-11.0615798711795));
#2190=CARTESIAN_POINT('Ctrl Pts',(7.88016511000832,40.6131682833795,-8.91948670360617));
#2191=CARTESIAN_POINT('Ctrl Pts',(7.66541391347513,40.6607235779339,-7.77929728029815));
#2192=CARTESIAN_POINT('Ctrl Pts',(6.79640351541145,40.8293540083924,-5.68538230247293));
#2193=CARTESIAN_POINT('Ctrl Pts',(6.14230817135067,40.9476179603983,-4.73136330668694));
#2194=CARTESIAN_POINT('Ctrl Pts',(4.63575860476114,41.1637585877487,-3.22580998516966));
#2195=CARTESIAN_POINT('Ctrl Pts',(3.68206578130104,41.2758539577384,-2.57252129598781));
#2196=CARTESIAN_POINT('Ctrl Pts',(1.5892054277245,41.4218020260498,-1.70479899207882));
#2197=CARTESIAN_POINT('Ctrl Pts',(0.449797224212467,41.4531912783312,-1.49053328739287));
#2198=CARTESIAN_POINT('Ctrl Pts',(-0.619834889991665,41.4359646982476,-1.49053328739287));
#2199=CARTESIAN_POINT('Origin',(27.9920812595258,-52.5591081221322,-29.9998965134939));
#2200=CARTESIAN_POINT('',(37.9920812595258,-52.5591081221322,10.0001034865061));
#2201=CARTESIAN_POINT('',(27.9920812595258,-52.5591081221322,10.0001034865061));
#2202=CARTESIAN_POINT('',(27.9920812595258,-52.5591081221322,10.0001034865061));
#2203=CARTESIAN_POINT('',(37.9920812595258,-52.5591081221322,-29.9998965134939));
#2204=CARTESIAN_POINT('',(37.9920812595258,-52.5591081221322,-29.9998965134939));
#2205=CARTESIAN_POINT('',(27.9920812595258,-52.5591081221322,-29.9998965134939));
#2206=CARTESIAN_POINT('',(27.9920812595258,-52.5591081221322,-29.9998965134939));
#2207=CARTESIAN_POINT('',(27.9920812595258,-52.5591081221322,-29.9998965134939));
#2208=CARTESIAN_POINT('Origin',(37.9920812595258,3.44089187786782,-29.9998965134939));
#2209=CARTESIAN_POINT('',(37.9920812595258,3.44089187786782,10.0001034865061));
#2210=CARTESIAN_POINT('',(37.9920812595258,3.44089187786782,10.0001034865061));
#2211=CARTESIAN_POINT('',(37.9920812595258,3.44089187786782,-29.9998965134939));
#2212=CARTESIAN_POINT('',(37.9920812595258,3.44089187786782,-29.9998965134939));
#2213=CARTESIAN_POINT('',(37.9920812595258,3.44089187786782,-29.9998965134939));
#2214=CARTESIAN_POINT('Origin',(-0.00791874047421016,3.44089187786782,-29.9998965134939));
#2215=CARTESIAN_POINT('',(-38.0079187404742,3.44089187786782,10.0001034865061));
#2216=CARTESIAN_POINT('Origin',(-0.00791874047421016,3.44089187786782,10.0001034865061));
#2217=CARTESIAN_POINT('',(-38.0079187404742,3.44089187786782,-29.9998965134939));
#2218=CARTESIAN_POINT('',(-38.0079187404742,3.44089187786782,-29.9998965134939));
#2219=CARTESIAN_POINT('Origin',(-0.00791874047421016,3.44089187786782,-29.9998965134939));
#2220=CARTESIAN_POINT('Origin',(-38.0079187404742,3.44089187786782,-29.9998965134939));
#2221=CARTESIAN_POINT('',(-38.0079187404742,-52.5591081221322,10.0001034865061));
#2222=CARTESIAN_POINT('',(-38.0079187404742,3.44089187786782,10.0001034865061));
#2223=CARTESIAN_POINT('',(-38.0079187404742,-52.5591081221322,-29.9998965134939));
#2224=CARTESIAN_POINT('',(-38.0079187404742,-52.5591081221322,-29.9998965134939));
#2225=CARTESIAN_POINT('',(-38.0079187404742,3.44089187786782,-29.9998965134939));
#2226=CARTESIAN_POINT('Origin',(-28.0079187404742,-52.5591081221322,-29.9998965134939));
#2227=CARTESIAN_POINT('',(-28.0079187404742,-52.5591081221322,10.0001034865061));
#2228=CARTESIAN_POINT('',(-28.0079187404742,-52.5591081221322,10.0001034865061));
#2229=CARTESIAN_POINT('',(-28.0079187404742,-52.5591081221322,-29.9998965134939));
#2230=CARTESIAN_POINT('',(-28.0079187404742,-52.5591081221322,-29.9998965134939));
#2231=CARTESIAN_POINT('',(-28.0079187404742,-52.5591081221322,-29.9998965134939));
#2232=CARTESIAN_POINT('Origin',(-28.0079187404742,-66.5591081221322,-29.9998965134939));
#2233=CARTESIAN_POINT('',(-28.0079187404742,-66.5591081221322,10.0001034865061));
#2234=CARTESIAN_POINT('',(-28.0079187404742,-66.5591081221322,10.0001034865061));
#2235=CARTESIAN_POINT('',(-28.0079187404742,-66.5591081221322,-29.9998965134939));
#2236=CARTESIAN_POINT('',(-28.0079187404742,-66.5591081221322,-29.9998965134939));
#2237=CARTESIAN_POINT('',(-28.0079187404742,-66.5591081221322,-29.9998965134939));
#2238=CARTESIAN_POINT('Origin',(-50.0079187404742,-66.5591081221322,-29.9998965134939));
#2239=CARTESIAN_POINT('',(-44.0079187404742,-66.5591081221322,10.0001034865061));
#2240=CARTESIAN_POINT('',(-50.0079187404742,-66.5591081221322,10.0001034865061));
#2241=CARTESIAN_POINT('',(-44.0079187404742,-66.5591081221322,-29.9998965134939));
#2242=CARTESIAN_POINT('',(-44.0079187404742,-66.5591081221322,-29.9998965134939));
#2243=CARTESIAN_POINT('',(-50.0079187404742,-66.5591081221322,-29.9998965134939));
#2244=CARTESIAN_POINT('Origin',(-50.0079187404742,3.44089187786782,-29.9998965134939));
#2245=CARTESIAN_POINT('',(-50.0079187404742,3.44089187786783,-29.9998965134939));
#2246=CARTESIAN_POINT('',(-50.0079187404742,-60.5591081221322,-29.9998965134939));
#2247=CARTESIAN_POINT('',(-50.0079187404742,3.44089187786782,-29.9998965134939));
#2248=CARTESIAN_POINT('',(-50.0079187404742,-60.5591081221322,10.0001034865061));
#2249=CARTESIAN_POINT('',(-50.0079187404742,-60.5591081221322,-29.9998965134939));
#2250=CARTESIAN_POINT('',(-50.0079187404742,3.44089187786783,10.0001034865061));
#2251=CARTESIAN_POINT('',(-50.0079187404742,3.44089187786782,10.0001034865061));
#2252=CARTESIAN_POINT('',(-50.0079187404742,3.44089187786783,-29.9998965134939));
#2253=CARTESIAN_POINT('Origin',(-0.00791874047421016,3.44089187786782,-29.9998965134939));
#2254=CARTESIAN_POINT('',(-18.7579187404742,49.7921324222157,10.0001034865061));
#2255=CARTESIAN_POINT('Origin',(-0.00791874047421016,3.44089187786782,10.0001034865061));
#2256=CARTESIAN_POINT('',(-18.7579187404742,49.7921324222157,-29.9998965134939));
#2257=CARTESIAN_POINT('',(-18.7579187404742,49.7921324222157,-29.9998965134939));
#2258=CARTESIAN_POINT('Origin',(-0.00791874047421016,3.44089187786782,-29.9998965134939));
#2259=CARTESIAN_POINT('Origin',(-15.0079187404742,57.4408918778678,-29.9998965134939));
#2260=CARTESIAN_POINT('',(-15.0079187404742,57.4408918778678,-29.9998965134939));
#2261=CARTESIAN_POINT('',(-15.0079187404742,55.3542812875375,-29.9998965134939));
#2262=CARTESIAN_POINT('',(-15.0079187404742,57.4408918778678,-29.9998965134939));
#2263=CARTESIAN_POINT('',(-15.0079187404742,55.3542812875375,10.0001034865061));
#2264=CARTESIAN_POINT('',(-15.0079187404742,55.3542812875375,10.0001034865061));
#2265=CARTESIAN_POINT('',(-15.0079187404742,57.4408918778678,10.0001034865061));
#2266=CARTESIAN_POINT('',(-15.0079187404742,57.4408918778678,10.0001034865061));
#2267=CARTESIAN_POINT('',(-15.0079187404742,57.4408918778678,-29.9998965134939));
#2268=CARTESIAN_POINT('Origin',(-0.00791874047421016,57.4408918778678,-29.9998965134939));
#2269=CARTESIAN_POINT('',(14.9920812595258,57.4408918778678,10.0001034865061));
#2270=CARTESIAN_POINT('',(-0.00791874047421016,57.4408918778678,10.0001034865061));
#2271=CARTESIAN_POINT('',(14.9920812595258,57.4408918778678,-29.9998965134939));
#2272=CARTESIAN_POINT('',(14.9920812595258,57.4408918778678,-29.9998965134939));
#2273=CARTESIAN_POINT('',(-0.00791874047421016,57.4408918778678,-29.9998965134939));
#2274=CARTESIAN_POINT('Origin',(14.9920812595258,57.4408918778678,-29.9998965134939));
#2275=CARTESIAN_POINT('',(14.9920812595258,55.3542812875375,10.0001034865061));
#2276=CARTESIAN_POINT('',(14.9920812595258,57.4408918778678,10.0001034865061));
#2277=CARTESIAN_POINT('',(14.9920812595258,55.3542812875375,-29.9998965134939));
#2278=CARTESIAN_POINT('',(14.9920812595258,55.3542812875375,-29.9998965134939));
#2279=CARTESIAN_POINT('',(14.9920812595258,57.4408918778678,-29.9998965134939));
#2280=CARTESIAN_POINT('Origin',(-0.00791874047421016,3.44089187786782,-29.9998965134939));
#2281=CARTESIAN_POINT('',(49.9920812595258,3.44089187786782,-29.9998965134939));
#2282=CARTESIAN_POINT('',(18.7420812595258,49.7921324222157,-29.9998965134939));
#2283=CARTESIAN_POINT('Origin',(-0.00791874047421016,3.44089187786782,-29.9998965134939));
#2284=CARTESIAN_POINT('',(18.7420812595258,49.7921324222157,10.0001034865061));
#2285=CARTESIAN_POINT('',(18.7420812595258,49.7921324222157,-29.9998965134939));
#2286=CARTESIAN_POINT('',(49.9920812595258,3.44089187786782,10.0001034865061));
#2287=CARTESIAN_POINT('Origin',(-0.00791874047421016,3.44089187786782,10.0001034865061));
#2288=CARTESIAN_POINT('',(49.9920812595258,3.44089187786782,-29.9998965134939));
#2289=CARTESIAN_POINT('Origin',(49.9920812595258,-66.5591081221322,-29.9998965134939));
#2290=CARTESIAN_POINT('',(49.9920812595258,-60.5591081221322,10.0001034865061));
#2291=CARTESIAN_POINT('',(49.9920812595258,-66.5591081221322,10.0001034865061));
#2292=CARTESIAN_POINT('',(49.9920812595258,-60.5591081221322,-29.9998965134939));
#2293=CARTESIAN_POINT('',(49.9920812595258,-60.5591081221322,-29.9998965134939));
#2294=CARTESIAN_POINT('',(49.9920812595258,-66.5591081221322,-29.9998965134939));
#2295=CARTESIAN_POINT('Origin',(49.9920812595258,-66.5591081221322,-29.9998965134939));
#2296=CARTESIAN_POINT('',(27.9920812595258,-66.5591081221322,-29.9998965134939));
#2297=CARTESIAN_POINT('',(43.9920812595258,-66.5591081221322,-29.9998965134939));
#2298=CARTESIAN_POINT('',(49.9920812595258,-66.5591081221322,-29.9998965134939));
#2299=CARTESIAN_POINT('',(43.9920812595258,-66.5591081221322,10.0001034865061));
#2300=CARTESIAN_POINT('',(43.9920812595258,-66.5591081221322,-29.9998965134939));
#2301=CARTESIAN_POINT('',(27.9920812595258,-66.5591081221322,10.0001034865061));
#2302=CARTESIAN_POINT('',(49.9920812595258,-66.5591081221322,10.0001034865061));
#2303=CARTESIAN_POINT('',(27.9920812595258,-66.5591081221322,-29.9998965134939));
#2304=CARTESIAN_POINT('Origin',(27.9920812595258,-66.5591081221322,-29.9998965134939));
#2305=CARTESIAN_POINT('',(27.9920812595258,-66.5591081221322,10.0001034865061));
#2306=CARTESIAN_POINT('',(27.9920812595258,-66.5591081221322,-29.9998965134939));
#2307=CARTESIAN_POINT('Origin',(-0.00791874047421016,3.44089187786782,-29.9998965134939));
#2308=CARTESIAN_POINT('Origin',(43.9920812595258,-60.5591081221322,-29.9998965134939));
#2309=CARTESIAN_POINT('Origin',(-44.0079187404742,-60.5591081221322,-29.9998965134939));
#2310=CARTESIAN_POINT('Origin',(-21.0079187404742,55.3542812875375,-29.9998965134939));
#2311=CARTESIAN_POINT('Origin',(20.9920812595258,55.3542812875375,-29.9998965134939));
#2312=CARTESIAN_POINT('Origin',(-0.00791874047421016,3.44089187786782,10.0001034865061));
#2313=CARTESIAN_POINT('Origin',(43.9920812595258,-60.5591081221322,10.0001034865061));
#2314=CARTESIAN_POINT('Origin',(20.9920812595258,55.3542812875375,10.0001034865061));
#2315=CARTESIAN_POINT('Origin',(-21.0079187404742,55.3542812875375,10.0001034865061));
#2316=CARTESIAN_POINT('Origin',(-44.0079187404742,-60.5591081221322,10.0001034865061));
#2317=CARTESIAN_POINT('Origin',(43.9920812595258,-60.5591081221322,-29.9998965134939));
#2318=CARTESIAN_POINT('Origin',(-44.0079187404742,-60.5591081221322,-29.9998965134939));
#2319=CARTESIAN_POINT('Origin',(-21.0079187404742,55.3542812875375,-29.9998965134939));
#2320=CARTESIAN_POINT('Origin',(20.9920812595258,55.3542812875375,-29.9998965134939));
#2468=UNCERTAINTY_MEASURE_WITH_UNIT(LENGTH_MEASURE(0.01),#2478,
'DISTANCE_ACCURACY_VALUE',
'Maximum model space distance between geometric entities at asserted c
onnectivities');
#2471=UNCERTAINTY_MEASURE_WITH_UNIT(LENGTH_MEASURE(0.01),#2478,
'DISTANCE_ACCURACY_VALUE',
'Maximum model space distance between geometric entities at asserted c
onnectivities');
#2474=(
GEOMETRIC_REPRESENTATION_CONTEXT(3)
GLOBAL_UNCERTAINTY_ASSIGNED_CONTEXT((#2468))
GLOBAL_UNIT_ASSIGNED_CONTEXT((#2478,#2480,#2481))
REPRESENTATION_CONTEXT('','3D')
);
#2477=(
GEOMETRIC_REPRESENTATION_CONTEXT(3)
GLOBAL_UNCERTAINTY_ASSIGNED_CONTEXT((#2471))
GLOBAL_UNIT_ASSIGNED_CONTEXT((#2478,#2480,#2481))
REPRESENTATION_CONTEXT('','3D')
);
#2478=(
LENGTH_UNIT()
NAMED_UNIT(*)
SI_UNIT(.MILLI.,.METRE.)
);
#2480=(
NAMED_UNIT(*)
PLANE_ANGLE_UNIT()
SI_UNIT($,.RADIAN.)
);
#2481=(
NAMED_UNIT(*)
SI_UNIT($,.STERADIAN.)
SOLID_ANGLE_UNIT()
);
#2484=SHAPE_DEFINITION_REPRESENTATION(#2489,#2498);
#2489=PRODUCT_DEFINITION_SHAPE('',$,#2504);
#2498=SHAPE_REPRESENTATION('',(#1506),#2474);
#2501=PRODUCT_DEFINITION_CONTEXT('part definition',#2518,'design');
#2504=PRODUCT_DEFINITION('Clamp','Clamp',#2509,#2501);
#2509=PRODUCT_DEFINITION_FORMATION('',$,#2522);
#2518=APPLICATION_CONTEXT(
'Core Data for Automotive Mechanical Design Process');
#2519=PRODUCT_CONTEXT('part definition',#2518,'mechanical');
#2522=PRODUCT('Clamp','Clamp',$,(#2519));
#2527=PRESENTATION_STYLE_ASSIGNMENT((#2532));
#2532=SURFACE_STYLE_USAGE(.BOTH.,#2537);
#2537=SURFACE_SIDE_STYLE('',(#2542));
#2542=SURFACE_STYLE_FILL_AREA(#2547);
#2547=FILL_AREA_STYLE('Opaque(61,176,222)',(#2552));
#2552=FILL_AREA_STYLE_COLOUR('Opaque(61,176,222)',#2557);
#2557=COLOUR_RGB('Opaque(61,176,222)',0.23921568627451,0.690196078431373,
0.870588235294118);
ENDSEC;
END-ISO-10303-21;
